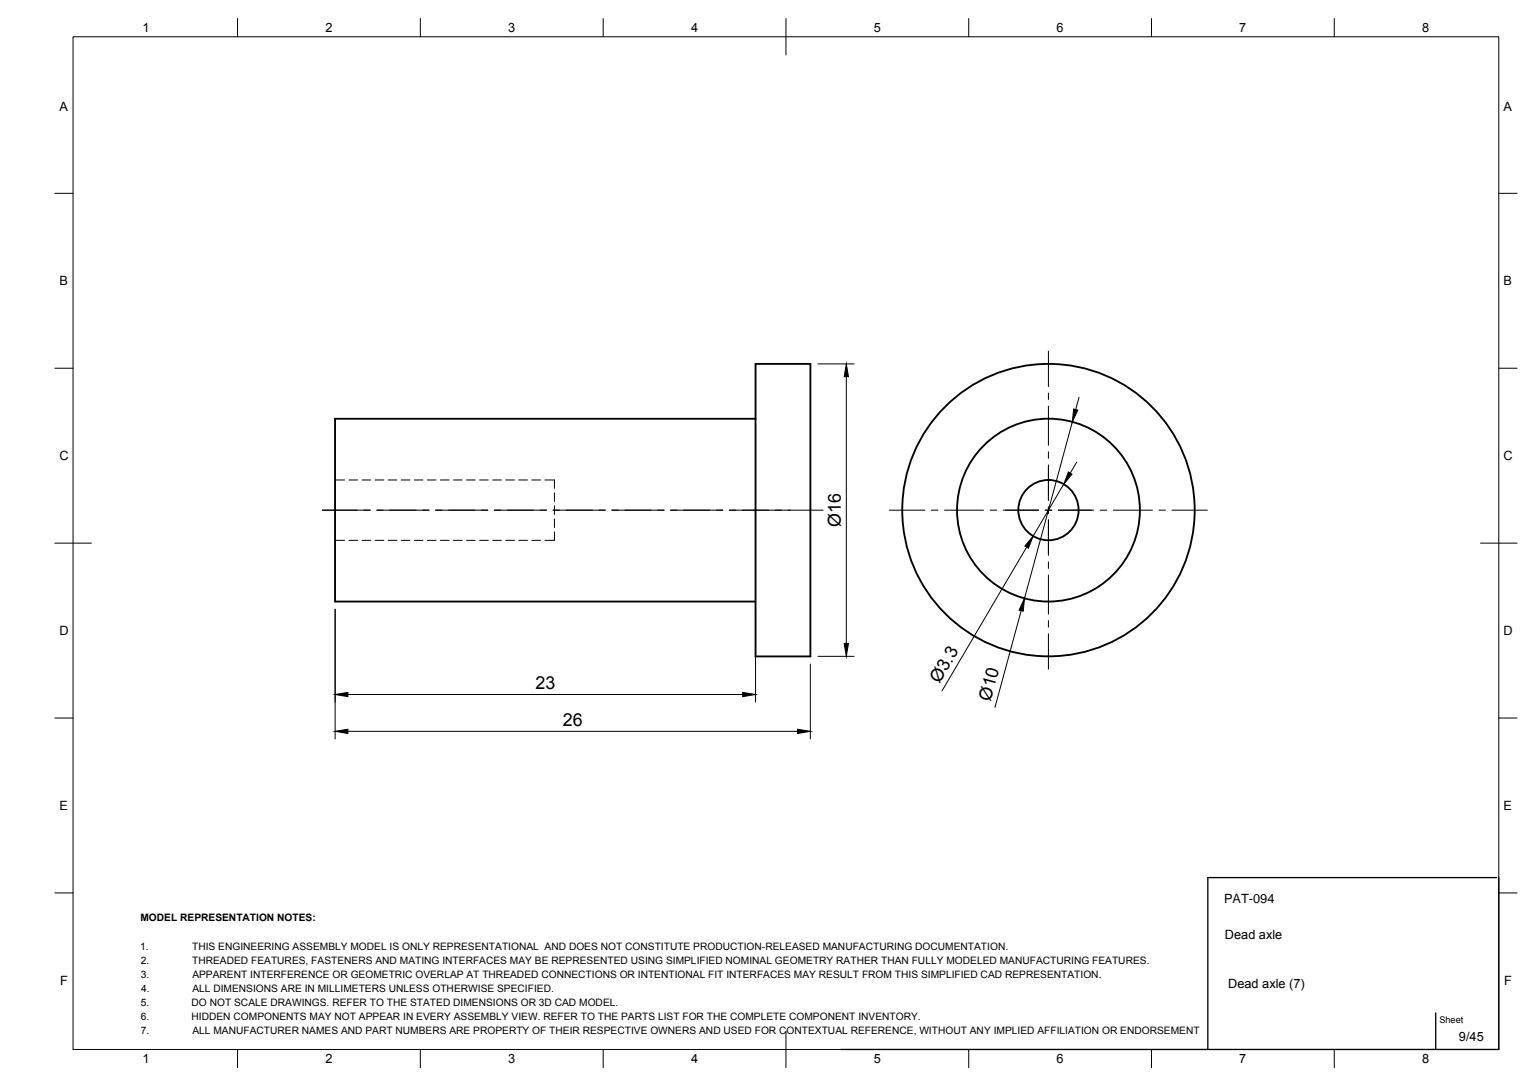
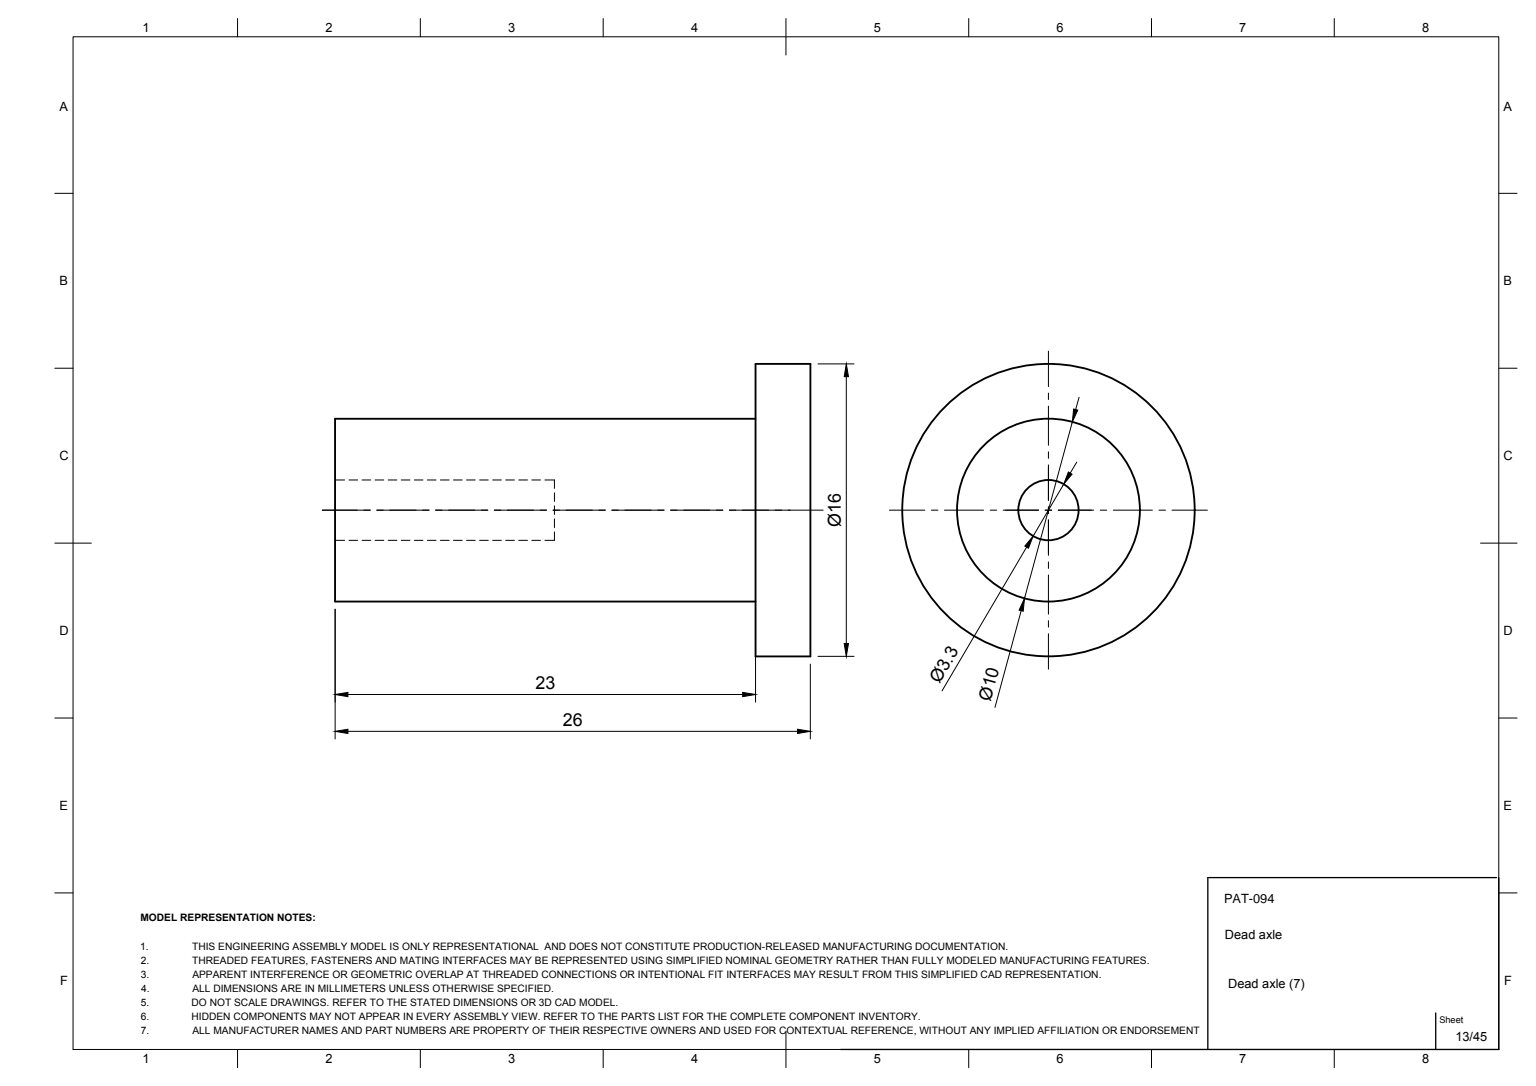
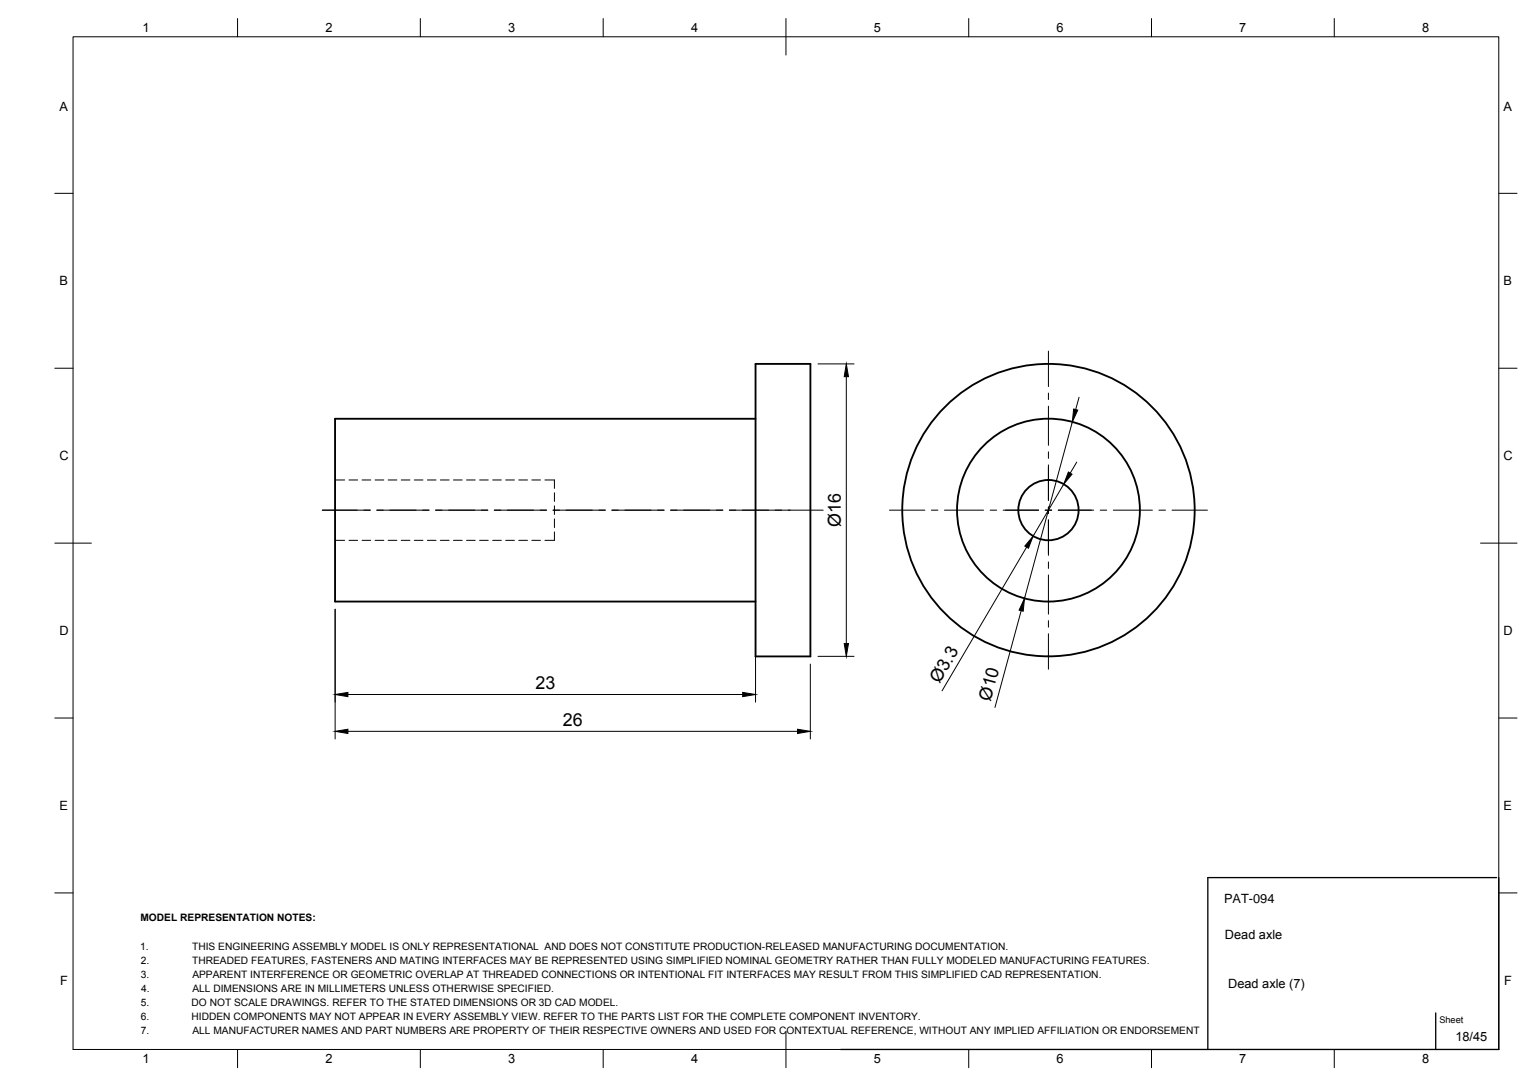
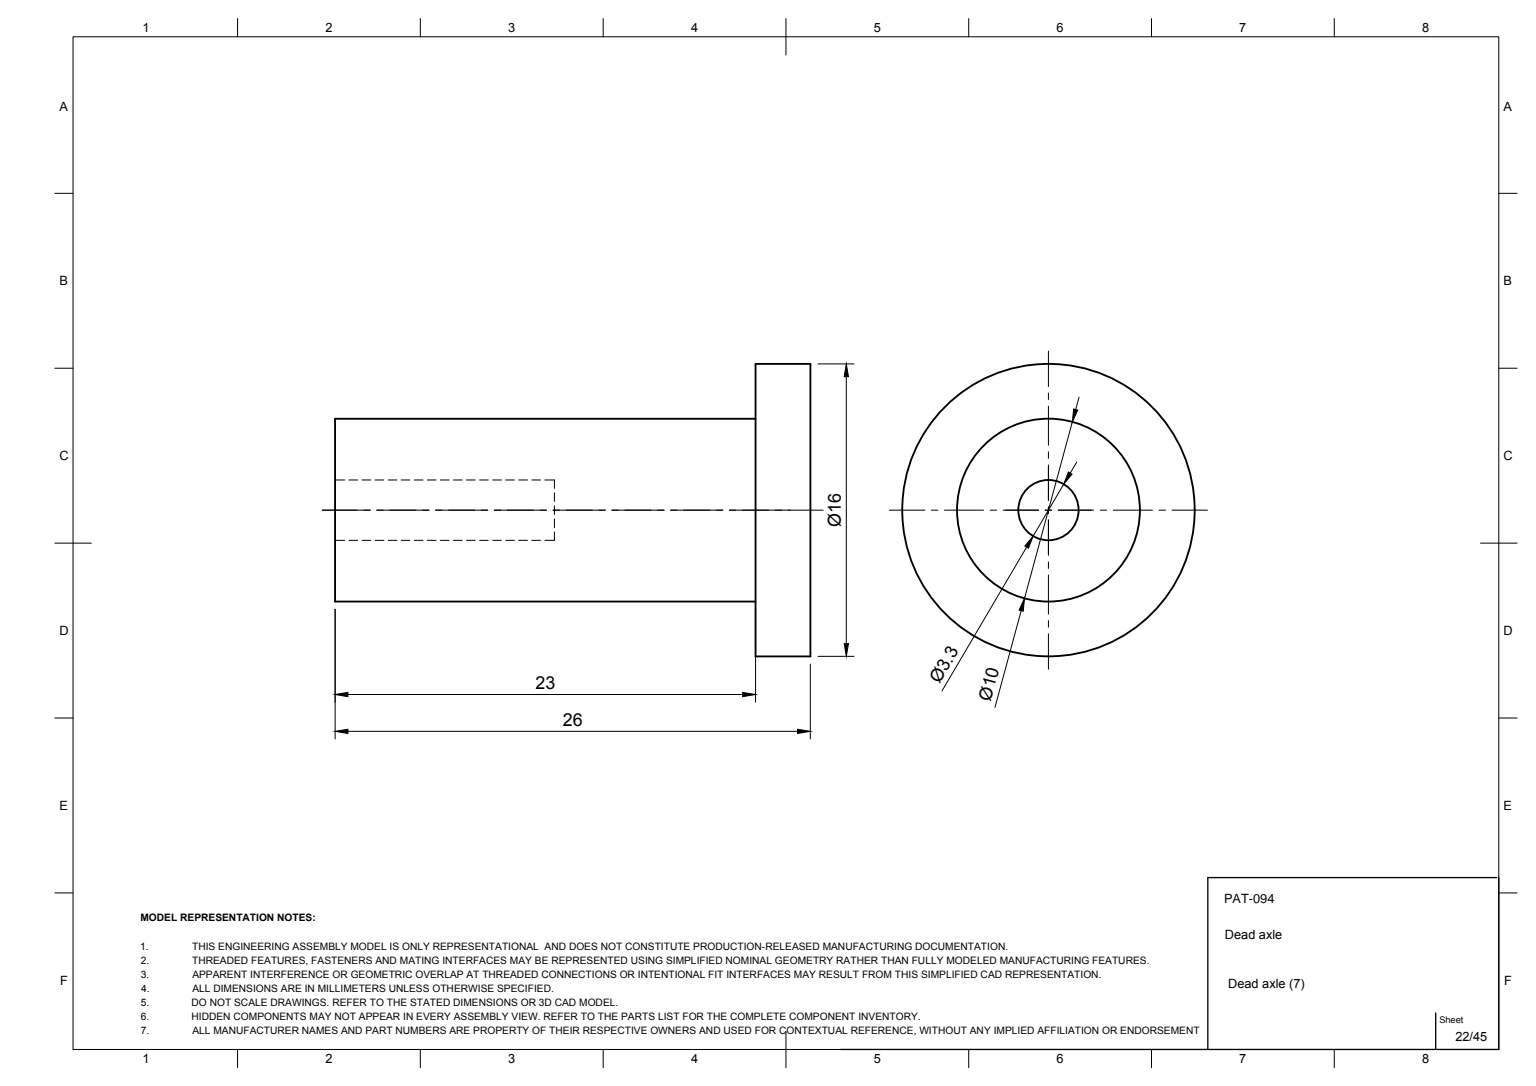
ISO-10303-21;
HEADER;
/* Generated by software containing ST-Developer
 * from STEP Tools, Inc. (www.steptools.com) 
 */

FILE_DESCRIPTION(
/* description */ ('Shaft runout checking stand'),
/* implementation_level */ '2;1');

FILE_NAME(
/* name */ 'Dead axle.step',
/* time_stamp */ '2026-11-02T21:12:33-08:00',
/* author */ (''),
/* organization */ (''),
/* preprocessor_version */ 'ST-DEVELOPER v20.2',
/* originating_system */ 'Autodesk Translation Framework v15.17.0.0',
/* authorisation */ '');

FILE_SCHEMA (('AUTOMOTIVE_DESIGN { 1 0 10303 214 3 1 1 }'));
ENDSEC;

DATA;
#10=MECHANICAL_DESIGN_GEOMETRIC_PRESENTATION_REPRESENTATION('',(#470),#11748);
#384=SHAPE_REPRESENTATION_RELATIONSHIP('SRR','None',#11933,#427);
#427=ADVANCED_BREP_SHAPE_REPRESENTATION('',(#521),#11709);
#470=STYLED_ITEM('',(#12169),#521);
#521=MANIFOLD_SOLID_BREP('Body1',#6213);
#599=FACE_BOUND('',#1556,.T.);
#600=FACE_BOUND('',#1561,.T.);
#718=CIRCLE('',#6902,0.165);
#719=CIRCLE('',#6903,0.165);
#720=CIRCLE('',#6906,0.8);
#721=CIRCLE('',#6907,0.5);
#722=CIRCLE('',#6909,0.8);
#723=CIRCLE('',#6912,0.5);
#959=CYLINDRICAL_SURFACE('',#6901,0.165);
#960=CYLINDRICAL_SURFACE('',#6908,0.8);
#961=CYLINDRICAL_SURFACE('',#6911,0.5);
#1148=FACE_OUTER_BOUND('',#1553,.T.);
#1149=FACE_OUTER_BOUND('',#1554,.T.);
#1150=FACE_OUTER_BOUND('',#1555,.T.);
#1151=FACE_OUTER_BOUND('',#1557,.T.);
#1152=FACE_OUTER_BOUND('',#1558,.T.);
#1153=FACE_OUTER_BOUND('',#1559,.T.);
#1154=FACE_OUTER_BOUND('',#1560,.T.);
#1553=EDGE_LOOP('',(#4668,#4669,#4670,#4671));
#1554=EDGE_LOOP('',(#4672));
#1555=EDGE_LOOP('',(#4673));
#1556=EDGE_LOOP('',(#4674));
#1557=EDGE_LOOP('',(#4675,#4676,#4677,#4678));
#1558=EDGE_LOOP('',(#4679));
#1559=EDGE_LOOP('',(#4680,#4681,#4682,#4683));
#1560=EDGE_LOOP('',(#4684));
#1561=EDGE_LOOP('',(#4685));
#2128=LINE('',#10082,#2595);
#2129=LINE('',#10092,#2596);
#2130=LINE('',#10098,#2597);
#2595=VECTOR('',#8073,0.165);
#2596=VECTOR('',#8086,0.8);
#2597=VECTOR('',#8095,0.5);
#3012=VERTEX_POINT('',#10079);
#3013=VERTEX_POINT('',#10081);
#3014=VERTEX_POINT('',#10086);
#3015=VERTEX_POINT('',#10088);
#3016=VERTEX_POINT('',#10091);
#3017=VERTEX_POINT('',#10096);
#3620=EDGE_CURVE('',#3012,#3012,#718,.T.);
#3621=EDGE_CURVE('',#3012,#3013,#2128,.T.);
#3622=EDGE_CURVE('',#3013,#3013,#719,.T.);
#3623=EDGE_CURVE('',#3014,#3014,#720,.T.);
#3624=EDGE_CURVE('',#3015,#3015,#721,.T.);
#3625=EDGE_CURVE('',#3014,#3016,#2129,.T.);
#3626=EDGE_CURVE('',#3016,#3016,#722,.T.);
#3627=EDGE_CURVE('',#3017,#3017,#723,.T.);
#3628=EDGE_CURVE('',#3017,#3015,#2130,.T.);
#4668=ORIENTED_EDGE('',*,*,#3620,.F.);
#4669=ORIENTED_EDGE('',*,*,#3621,.T.);
#4670=ORIENTED_EDGE('',*,*,#3622,.F.);
#4671=ORIENTED_EDGE('',*,*,#3621,.F.);
#4672=ORIENTED_EDGE('',*,*,#3620,.T.);
#4673=ORIENTED_EDGE('',*,*,#3623,.T.);
#4674=ORIENTED_EDGE('',*,*,#3624,.F.);
#4675=ORIENTED_EDGE('',*,*,#3623,.F.);
#4676=ORIENTED_EDGE('',*,*,#3625,.T.);
#4677=ORIENTED_EDGE('',*,*,#3626,.T.);
#4678=ORIENTED_EDGE('',*,*,#3625,.F.);
#4679=ORIENTED_EDGE('',*,*,#3626,.F.);
#4680=ORIENTED_EDGE('',*,*,#3627,.F.);
#4681=ORIENTED_EDGE('',*,*,#3628,.T.);
#4682=ORIENTED_EDGE('',*,*,#3624,.T.);
#4683=ORIENTED_EDGE('',*,*,#3628,.F.);
#4684=ORIENTED_EDGE('',*,*,#3627,.T.);
#4685=ORIENTED_EDGE('',*,*,#3622,.T.);
#5692=PLANE('',#6904);
#5693=PLANE('',#6905);
#5694=PLANE('',#6910);
#5695=PLANE('',#6913);
#5948=ADVANCED_FACE('',(#1148),#959,.F.);
#5949=ADVANCED_FACE('',(#1149),#5692,.T.);
#5950=ADVANCED_FACE('',(#1150,#599),#5693,.T.);
#5951=ADVANCED_FACE('',(#1151),#960,.T.);
#5952=ADVANCED_FACE('',(#1152),#5694,.F.);
#5953=ADVANCED_FACE('',(#1153),#961,.T.);
#5954=ADVANCED_FACE('',(#1154,#600),#5695,.T.);
#6213=CLOSED_SHELL('',(#5948,#5949,#5950,#5951,#5952,#5953,#5954));
#6900=AXIS2_PLACEMENT_3D('',#10077,#8067,#8068);
#6901=AXIS2_PLACEMENT_3D('',#10078,#8069,#8070);
#6902=AXIS2_PLACEMENT_3D('',#10080,#8071,#8072);
#6903=AXIS2_PLACEMENT_3D('',#10083,#8074,#8075);
#6904=AXIS2_PLACEMENT_3D('',#10084,#8076,#8077);
#6905=AXIS2_PLACEMENT_3D('',#10085,#8078,#8079);
#6906=AXIS2_PLACEMENT_3D('',#10087,#8080,#8081);
#6907=AXIS2_PLACEMENT_3D('',#10089,#8082,#8083);
#6908=AXIS2_PLACEMENT_3D('',#10090,#8084,#8085);
#6909=AXIS2_PLACEMENT_3D('',#10093,#8087,#8088);
#6910=AXIS2_PLACEMENT_3D('',#10094,#8089,#8090);
#6911=AXIS2_PLACEMENT_3D('',#10095,#8091,#8092);
#6912=AXIS2_PLACEMENT_3D('',#10097,#8093,#8094);
#6913=AXIS2_PLACEMENT_3D('',#10099,#8096,#8097);
#8067=DIRECTION('axis',(0.,0.,1.));
#8068=DIRECTION('refdir',(1.,0.,0.));
#8069=DIRECTION('center_axis',(0.,1.,0.));
#8070=DIRECTION('ref_axis',(1.,0.,0.));
#8071=DIRECTION('center_axis',(0.,1.,0.));
#8072=DIRECTION('ref_axis',(1.,0.,0.));
#8073=DIRECTION('',(0.,1.,0.));
#8074=DIRECTION('center_axis',(0.,-1.,0.));
#8075=DIRECTION('ref_axis',(1.,0.,0.));
#8076=DIRECTION('center_axis',(0.,1.,0.));
#8077=DIRECTION('ref_axis',(1.,0.,0.));
#8078=DIRECTION('center_axis',(0.,1.,0.));
#8079=DIRECTION('ref_axis',(1.,0.,0.));
#8080=DIRECTION('center_axis',(0.,1.,0.));
#8081=DIRECTION('ref_axis',(1.,0.,0.));
#8082=DIRECTION('center_axis',(0.,1.,0.));
#8083=DIRECTION('ref_axis',(1.,0.,0.));
#8084=DIRECTION('center_axis',(0.,1.,0.));
#8085=DIRECTION('ref_axis',(1.,0.,0.));
#8086=DIRECTION('',(0.,-1.,0.));
#8087=DIRECTION('center_axis',(0.,1.,0.));
#8088=DIRECTION('ref_axis',(1.,0.,0.));
#8089=DIRECTION('center_axis',(0.,1.,0.));
#8090=DIRECTION('ref_axis',(1.,0.,0.));
#8091=DIRECTION('center_axis',(0.,1.,0.));
#8092=DIRECTION('ref_axis',(1.,0.,0.));
#8093=DIRECTION('center_axis',(0.,1.,0.));
#8094=DIRECTION('ref_axis',(1.,0.,0.));
#8095=DIRECTION('',(0.,-1.,0.));
#8096=DIRECTION('center_axis',(0.,1.,0.));
#8097=DIRECTION('ref_axis',(1.,0.,0.));
#10077=CARTESIAN_POINT('',(0.,0.,0.));
#10078=CARTESIAN_POINT('Origin',(-2.,-10.4,5.));
#10079=CARTESIAN_POINT('',(-2.165,-10.4,5.));
#10080=CARTESIAN_POINT('Origin',(-2.,-10.4,5.));
#10081=CARTESIAN_POINT('',(-2.165,-9.2,5.));
#10082=CARTESIAN_POINT('',(-2.165,-10.4,5.));
#10083=CARTESIAN_POINT('Origin',(-2.,-9.2,5.));
#10084=CARTESIAN_POINT('Origin',(-2.,-10.4,5.));
#10085=CARTESIAN_POINT('Origin',(-2.,-11.5,5.));
#10086=CARTESIAN_POINT('',(-2.8,-11.5,5.));
#10087=CARTESIAN_POINT('Origin',(-2.,-11.5,5.));
#10088=CARTESIAN_POINT('',(-2.5,-11.5,5.));
#10089=CARTESIAN_POINT('Origin',(-2.,-11.5,5.));
#10090=CARTESIAN_POINT('Origin',(-2.,-11.8,5.));
#10091=CARTESIAN_POINT('',(-2.8,-11.8,5.));
#10092=CARTESIAN_POINT('',(-2.8,-11.8,5.));
#10093=CARTESIAN_POINT('Origin',(-2.,-11.8,5.));
#10094=CARTESIAN_POINT('Origin',(-2.,-11.8,5.));
#10095=CARTESIAN_POINT('Origin',(-2.,-11.5,5.));
#10096=CARTESIAN_POINT('',(-2.5,-9.2,5.));
#10097=CARTESIAN_POINT('Origin',(-2.,-9.2,5.));
#10098=CARTESIAN_POINT('',(-2.5,-11.5,5.));
#10099=CARTESIAN_POINT('Origin',(-2.,-9.2,5.));
#11660=UNCERTAINTY_MEASURE_WITH_UNIT(LENGTH_MEASURE(0.001),#11749,
'DISTANCE_ACCURACY_VALUE',
'Maximum model space distance between geometric entities at asserted c
onnectivities');
#11699=UNCERTAINTY_MEASURE_WITH_UNIT(LENGTH_MEASURE(0.001),#11749,
'DISTANCE_ACCURACY_VALUE',
'Maximum model space distance between geometric entities at asserted c
onnectivities');
#11709=(
GEOMETRIC_REPRESENTATION_CONTEXT(3)
GLOBAL_UNCERTAINTY_ASSIGNED_CONTEXT((#11660))
GLOBAL_UNIT_ASSIGNED_CONTEXT((#11749,#11751,#11752))
REPRESENTATION_CONTEXT('','3D')
);
#11748=(
GEOMETRIC_REPRESENTATION_CONTEXT(3)
GLOBAL_UNCERTAINTY_ASSIGNED_CONTEXT((#11699))
GLOBAL_UNIT_ASSIGNED_CONTEXT((#11749,#11751,#11752))
REPRESENTATION_CONTEXT('','3D')
);
#11749=(
LENGTH_UNIT()
NAMED_UNIT(*)
SI_UNIT(.CENTI.,.METRE.)
);
#11751=(
NAMED_UNIT(*)
PLANE_ANGLE_UNIT()
SI_UNIT($,.RADIAN.)
);
#11752=(
NAMED_UNIT(*)
SI_UNIT($,.STERADIAN.)
SOLID_ANGLE_UNIT()
);
#11762=SHAPE_DEFINITION_REPRESENTATION(#11810,#11933);
#11810=PRODUCT_DEFINITION_SHAPE('',$,#11982);
#11933=SHAPE_REPRESENTATION('',(#6900),#11709);
#11972=PRODUCT_DEFINITION_CONTEXT('part definition',#12118,'design');
#11982=PRODUCT_DEFINITION('Dead axle','Dead axle',#12030,#11972);
#12030=PRODUCT_DEFINITION_FORMATION('',$,#12129);
#12118=APPLICATION_CONTEXT(
'Core Data for Automotive Mechanical Design Process');
#12119=PRODUCT_CONTEXT('part definition',#12118,'mechanical');
#12129=PRODUCT('Dead axle','Dead axle','Dead axle',(#12119));
#12169=PRESENTATION_STYLE_ASSIGNMENT((#12174));
#12174=SURFACE_STYLE_USAGE(.BOTH.,#12179);
#12179=SURFACE_SIDE_STYLE('',(#12184));
#12184=SURFACE_STYLE_FILL_AREA(#12189);
#12189=FILL_AREA_STYLE('CAD Library Painted - Engineering blue',(#12194));
#12194=FILL_AREA_STYLE_COLOUR('CAD Library Painted - Engineering blue',
#12199);
#12199=COLOUR_RGB('CAD Library Painted - Engineering blue',0.12156862745098,
0.356862745098039,0.6);
ENDSEC;
END-ISO-10303-21;
